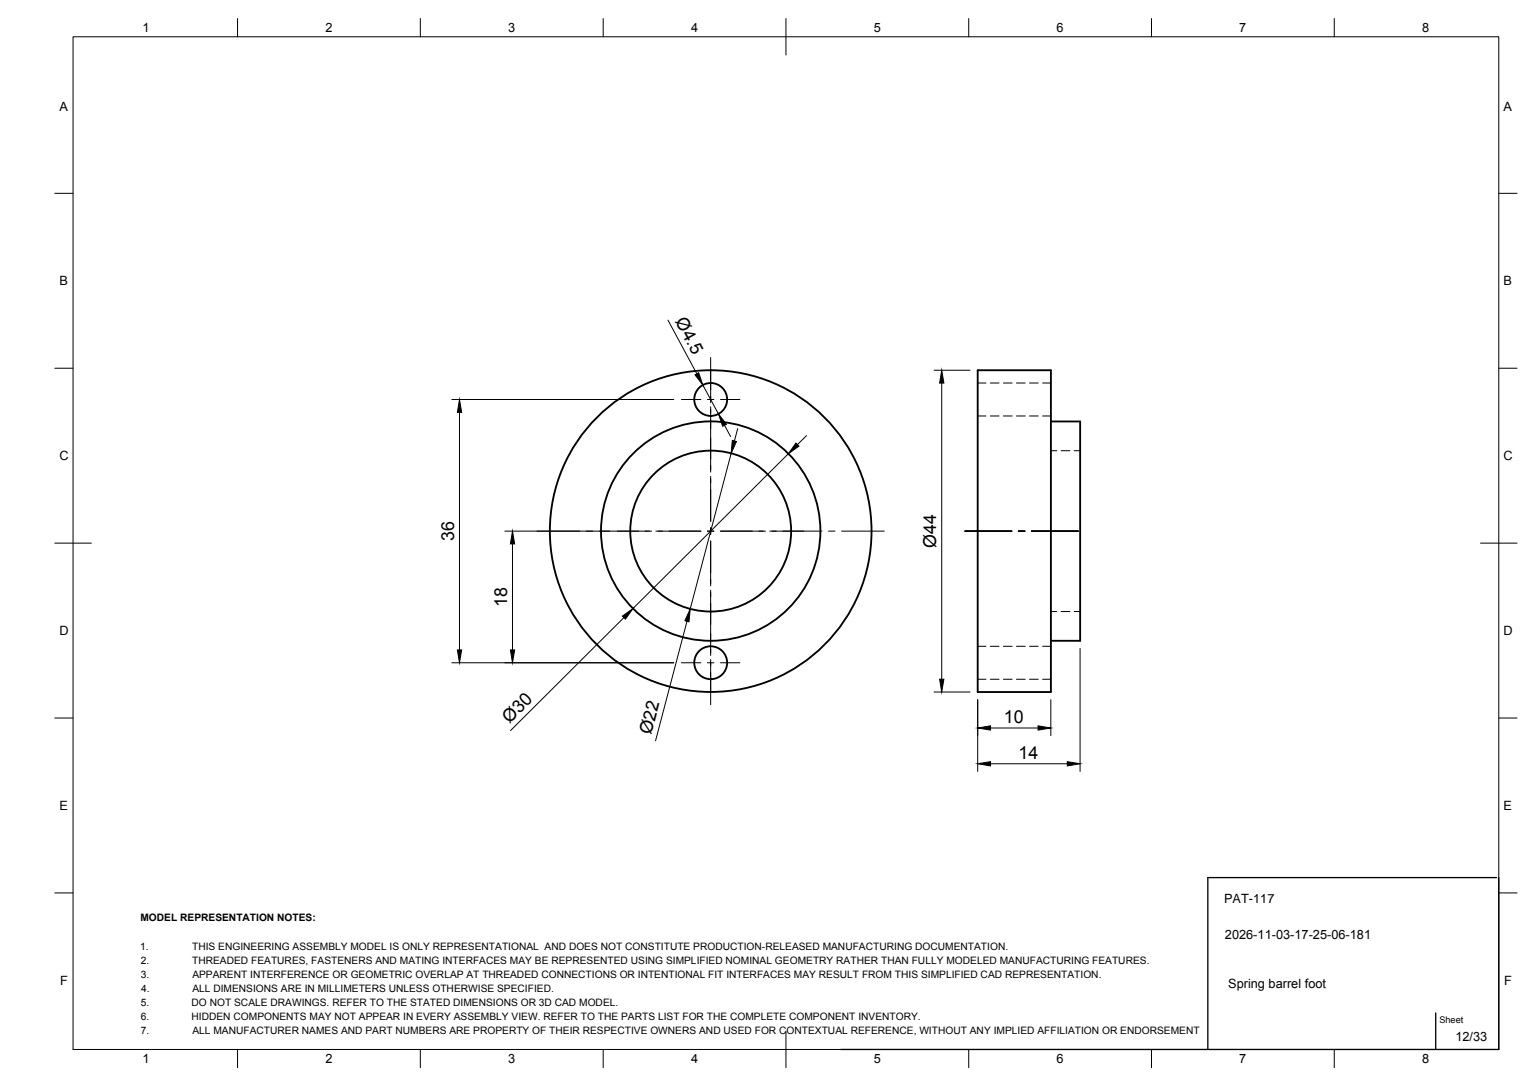
ISO-10303-21;
HEADER;
/* Generated by software containing ST-Developer
 * from STEP Tools, Inc. (www.steptools.com) 
 */

FILE_DESCRIPTION(
/* description */ ('Counterbalanced vertical column'),
/* implementation_level */ '2;1');

FILE_NAME(
/* name */ 'Spring barrel foot.step',
/* time_stamp */ '2026-10-29T16:47:22-07:00',
/* author */ (''),
/* organization */ (''),
/* preprocessor_version */ 'ST-DEVELOPER v20.2',
/* originating_system */ 'Autodesk Translation Framework v15.17.0.0',
/* authorisation */ '');

FILE_SCHEMA (('AUTOMOTIVE_DESIGN { 1 0 10303 214 3 1 1 }'));
ENDSEC;

DATA;
#10=MECHANICAL_DESIGN_GEOMETRIC_PRESENTATION_REPRESENTATION('',(#357),#15040);
#287=SHAPE_REPRESENTATION_RELATIONSHIP('SRR','None',#15191,#322);
#322=ADVANCED_BREP_SHAPE_REPRESENTATION('',(#392),#15010);
#357=STYLED_ITEM('',(#15457),#392);
#392=MANIFOLD_SOLID_BREP('Body1',#7080);
#444=FACE_BOUND('',#1330,.T.);
#445=FACE_BOUND('',#1332,.T.);
#446=FACE_BOUND('',#1333,.T.);
#447=FACE_BOUND('',#1334,.T.);
#448=FACE_BOUND('',#1338,.T.);
#449=FACE_BOUND('',#1339,.T.);
#581=PLANE('',#7618);
#582=PLANE('',#7619);
#583=PLANE('',#7623);
#584=PLANE('',#7624);
#892=FACE_OUTER_BOUND('',#1325,.T.);
#893=FACE_OUTER_BOUND('',#1326,.T.);
#894=FACE_OUTER_BOUND('',#1327,.T.);
#895=FACE_OUTER_BOUND('',#1328,.T.);
#896=FACE_OUTER_BOUND('',#1329,.T.);
#897=FACE_OUTER_BOUND('',#1331,.T.);
#898=FACE_OUTER_BOUND('',#1335,.T.);
#899=FACE_OUTER_BOUND('',#1336,.T.);
#900=FACE_OUTER_BOUND('',#1337,.T.);
#1325=EDGE_LOOP('',(#5076,#5077,#5078,#5079));
#1326=EDGE_LOOP('',(#5080,#5081,#5082,#5083));
#1327=EDGE_LOOP('',(#5084,#5085,#5086,#5087));
#1328=EDGE_LOOP('',(#5088,#5089,#5090,#5091));
#1329=EDGE_LOOP('',(#5092));
#1330=EDGE_LOOP('',(#5093));
#1331=EDGE_LOOP('',(#5094));
#1332=EDGE_LOOP('',(#5095));
#1333=EDGE_LOOP('',(#5096));
#1334=EDGE_LOOP('',(#5097));
#1335=EDGE_LOOP('',(#5098,#5099,#5100,#5101));
#1336=EDGE_LOOP('',(#5102));
#1337=EDGE_LOOP('',(#5103));
#1338=EDGE_LOOP('',(#5104));
#1339=EDGE_LOOP('',(#5105));
#1863=LINE('',#10658,#2534);
#1864=LINE('',#10664,#2535);
#1865=LINE('',#10670,#2536);
#1866=LINE('',#10676,#2537);
#1867=LINE('',#10684,#2538);
#2534=VECTOR('',#8553,0.225);
#2535=VECTOR('',#8560,0.225);
#2536=VECTOR('',#8567,1.1);
#2537=VECTOR('',#8574,1.5);
#2538=VECTOR('',#8585,2.2);
#3125=CIRCLE('',#7607,0.225);
#3126=CIRCLE('',#7608,0.225);
#3127=CIRCLE('',#7610,0.225);
#3128=CIRCLE('',#7611,0.225);
#3129=CIRCLE('',#7613,1.1);
#3130=CIRCLE('',#7614,1.1);
#3131=CIRCLE('',#7616,1.5);
#3132=CIRCLE('',#7617,1.5);
#3133=CIRCLE('',#7620,2.2);
#3134=CIRCLE('',#7622,2.2);
#3402=VERTEX_POINT('',#10655);
#3403=VERTEX_POINT('',#10657);
#3404=VERTEX_POINT('',#10661);
#3405=VERTEX_POINT('',#10663);
#3406=VERTEX_POINT('',#10667);
#3407=VERTEX_POINT('',#10669);
#3408=VERTEX_POINT('',#10673);
#3409=VERTEX_POINT('',#10675);
#3410=VERTEX_POINT('',#10680);
#3411=VERTEX_POINT('',#10683);
#4039=EDGE_CURVE('',#3402,#3402,#3125,.T.);
#4040=EDGE_CURVE('',#3402,#3403,#1863,.T.);
#4041=EDGE_CURVE('',#3403,#3403,#3126,.T.);
#4042=EDGE_CURVE('',#3404,#3404,#3127,.T.);
#4043=EDGE_CURVE('',#3404,#3405,#1864,.T.);
#4044=EDGE_CURVE('',#3405,#3405,#3128,.T.);
#4045=EDGE_CURVE('',#3406,#3406,#3129,.T.);
#4046=EDGE_CURVE('',#3406,#3407,#1865,.T.);
#4047=EDGE_CURVE('',#3407,#3407,#3130,.T.);
#4048=EDGE_CURVE('',#3408,#3408,#3131,.T.);
#4049=EDGE_CURVE('',#3408,#3409,#1866,.T.);
#4050=EDGE_CURVE('',#3409,#3409,#3132,.T.);
#4051=EDGE_CURVE('',#3410,#3410,#3133,.T.);
#4052=EDGE_CURVE('',#3410,#3411,#1867,.T.);
#4053=EDGE_CURVE('',#3411,#3411,#3134,.T.);
#5076=ORIENTED_EDGE('',*,*,#4039,.F.);
#5077=ORIENTED_EDGE('',*,*,#4040,.T.);
#5078=ORIENTED_EDGE('',*,*,#4041,.F.);
#5079=ORIENTED_EDGE('',*,*,#4040,.F.);
#5080=ORIENTED_EDGE('',*,*,#4042,.F.);
#5081=ORIENTED_EDGE('',*,*,#4043,.T.);
#5082=ORIENTED_EDGE('',*,*,#4044,.F.);
#5083=ORIENTED_EDGE('',*,*,#4043,.F.);
#5084=ORIENTED_EDGE('',*,*,#4045,.F.);
#5085=ORIENTED_EDGE('',*,*,#4046,.T.);
#5086=ORIENTED_EDGE('',*,*,#4047,.F.);
#5087=ORIENTED_EDGE('',*,*,#4046,.F.);
#5088=ORIENTED_EDGE('',*,*,#4048,.F.);
#5089=ORIENTED_EDGE('',*,*,#4049,.T.);
#5090=ORIENTED_EDGE('',*,*,#4050,.F.);
#5091=ORIENTED_EDGE('',*,*,#4049,.F.);
#5092=ORIENTED_EDGE('',*,*,#4048,.T.);
#5093=ORIENTED_EDGE('',*,*,#4045,.T.);
#5094=ORIENTED_EDGE('',*,*,#4051,.T.);
#5095=ORIENTED_EDGE('',*,*,#4041,.T.);
#5096=ORIENTED_EDGE('',*,*,#4044,.T.);
#5097=ORIENTED_EDGE('',*,*,#4050,.T.);
#5098=ORIENTED_EDGE('',*,*,#4051,.F.);
#5099=ORIENTED_EDGE('',*,*,#4052,.T.);
#5100=ORIENTED_EDGE('',*,*,#4053,.T.);
#5101=ORIENTED_EDGE('',*,*,#4052,.F.);
#5102=ORIENTED_EDGE('',*,*,#4047,.T.);
#5103=ORIENTED_EDGE('',*,*,#4053,.F.);
#5104=ORIENTED_EDGE('',*,*,#4039,.T.);
#5105=ORIENTED_EDGE('',*,*,#4042,.T.);
#6590=CYLINDRICAL_SURFACE('',#7606,0.225);
#6591=CYLINDRICAL_SURFACE('',#7609,0.225);
#6592=CYLINDRICAL_SURFACE('',#7612,1.1);
#6593=CYLINDRICAL_SURFACE('',#7615,1.5);
#6594=CYLINDRICAL_SURFACE('',#7621,2.2);
#6734=ADVANCED_FACE('',(#892),#6590,.F.);
#6735=ADVANCED_FACE('',(#893),#6591,.F.);
#6736=ADVANCED_FACE('',(#894),#6592,.F.);
#6737=ADVANCED_FACE('',(#895),#6593,.T.);
#6738=ADVANCED_FACE('',(#896,#444),#581,.T.);
#6739=ADVANCED_FACE('',(#897,#445,#446,#447),#582,.T.);
#6740=ADVANCED_FACE('',(#898),#6594,.T.);
#6741=ADVANCED_FACE('',(#899),#583,.T.);
#6742=ADVANCED_FACE('',(#900,#448,#449),#584,.F.);
#7080=CLOSED_SHELL('',(#6734,#6735,#6736,#6737,#6738,#6739,#6740,#6741,
#6742));
#7605=AXIS2_PLACEMENT_3D('',#10653,#8547,#8548);
#7606=AXIS2_PLACEMENT_3D('',#10654,#8549,#8550);
#7607=AXIS2_PLACEMENT_3D('',#10656,#8551,#8552);
#7608=AXIS2_PLACEMENT_3D('',#10659,#8554,#8555);
#7609=AXIS2_PLACEMENT_3D('',#10660,#8556,#8557);
#7610=AXIS2_PLACEMENT_3D('',#10662,#8558,#8559);
#7611=AXIS2_PLACEMENT_3D('',#10665,#8561,#8562);
#7612=AXIS2_PLACEMENT_3D('',#10666,#8563,#8564);
#7613=AXIS2_PLACEMENT_3D('',#10668,#8565,#8566);
#7614=AXIS2_PLACEMENT_3D('',#10671,#8568,#8569);
#7615=AXIS2_PLACEMENT_3D('',#10672,#8570,#8571);
#7616=AXIS2_PLACEMENT_3D('',#10674,#8572,#8573);
#7617=AXIS2_PLACEMENT_3D('',#10677,#8575,#8576);
#7618=AXIS2_PLACEMENT_3D('',#10678,#8577,#8578);
#7619=AXIS2_PLACEMENT_3D('',#10679,#8579,#8580);
#7620=AXIS2_PLACEMENT_3D('',#10681,#8581,#8582);
#7621=AXIS2_PLACEMENT_3D('',#10682,#8583,#8584);
#7622=AXIS2_PLACEMENT_3D('',#10685,#8586,#8587);
#7623=AXIS2_PLACEMENT_3D('',#10686,#8588,#8589);
#7624=AXIS2_PLACEMENT_3D('',#10687,#8590,#8591);
#8547=DIRECTION('axis',(0.,0.,1.));
#8548=DIRECTION('refdir',(1.,0.,0.));
#8549=DIRECTION('center_axis',(0.,0.,1.));
#8550=DIRECTION('ref_axis',(1.,0.,0.));
#8551=DIRECTION('center_axis',(0.,0.,1.));
#8552=DIRECTION('ref_axis',(1.,0.,0.));
#8553=DIRECTION('',(0.,0.,1.));
#8554=DIRECTION('center_axis',(0.,0.,-1.));
#8555=DIRECTION('ref_axis',(1.,0.,0.));
#8556=DIRECTION('center_axis',(0.,0.,1.));
#8557=DIRECTION('ref_axis',(1.,0.,0.));
#8558=DIRECTION('center_axis',(0.,0.,1.));
#8559=DIRECTION('ref_axis',(1.,0.,0.));
#8560=DIRECTION('',(0.,0.,1.));
#8561=DIRECTION('center_axis',(0.,0.,-1.));
#8562=DIRECTION('ref_axis',(1.,0.,0.));
#8563=DIRECTION('center_axis',(0.,0.,1.));
#8564=DIRECTION('ref_axis',(1.,0.,0.));
#8565=DIRECTION('center_axis',(0.,0.,-1.));
#8566=DIRECTION('ref_axis',(1.,0.,0.));
#8567=DIRECTION('',(0.,0.,-1.));
#8568=DIRECTION('center_axis',(0.,0.,1.));
#8569=DIRECTION('ref_axis',(1.,0.,0.));
#8570=DIRECTION('center_axis',(0.,0.,1.));
#8571=DIRECTION('ref_axis',(1.,0.,0.));
#8572=DIRECTION('center_axis',(0.,0.,1.));
#8573=DIRECTION('ref_axis',(1.,0.,0.));
#8574=DIRECTION('',(0.,0.,-1.));
#8575=DIRECTION('center_axis',(0.,0.,-1.));
#8576=DIRECTION('ref_axis',(1.,0.,0.));
#8577=DIRECTION('center_axis',(0.,0.,1.));
#8578=DIRECTION('ref_axis',(1.,0.,0.));
#8579=DIRECTION('center_axis',(0.,0.,1.));
#8580=DIRECTION('ref_axis',(1.,0.,0.));
#8581=DIRECTION('center_axis',(0.,0.,1.));
#8582=DIRECTION('ref_axis',(1.,0.,0.));
#8583=DIRECTION('center_axis',(0.,0.,1.));
#8584=DIRECTION('ref_axis',(1.,0.,0.));
#8585=DIRECTION('',(0.,0.,-1.));
#8586=DIRECTION('center_axis',(0.,0.,1.));
#8587=DIRECTION('ref_axis',(1.,0.,0.));
#8588=DIRECTION('center_axis',(0.,0.,1.));
#8589=DIRECTION('ref_axis',(1.,0.,0.));
#8590=DIRECTION('center_axis',(0.,0.,1.));
#8591=DIRECTION('ref_axis',(1.,0.,0.));
#10653=CARTESIAN_POINT('',(0.,0.,0.));
#10654=CARTESIAN_POINT('Origin',(-5.2,0.,-0.1));
#10655=CARTESIAN_POINT('',(-5.425,-2.75545529808154E-17,0.));
#10656=CARTESIAN_POINT('Origin',(-5.2,0.,0.));
#10657=CARTESIAN_POINT('',(-5.425,2.75545529808154E-17,1.));
#10658=CARTESIAN_POINT('',(-5.425,-2.75545529808154E-17,-0.1));
#10659=CARTESIAN_POINT('Origin',(-5.2,0.,1.));
#10660=CARTESIAN_POINT('Origin',(-8.8,0.,-0.1));
#10661=CARTESIAN_POINT('',(-9.025,-2.75545529808154E-17,0.));
#10662=CARTESIAN_POINT('Origin',(-8.8,0.,0.));
#10663=CARTESIAN_POINT('',(-9.025,2.75545529808154E-17,1.));
#10664=CARTESIAN_POINT('',(-9.025,-2.75545529808154E-17,-0.1));
#10665=CARTESIAN_POINT('Origin',(-8.8,0.,1.));
#10666=CARTESIAN_POINT('Origin',(-7.,0.,1.));
#10667=CARTESIAN_POINT('',(-8.1,-1.34711147906209E-16,1.4));
#10668=CARTESIAN_POINT('Origin',(-7.,0.,1.4));
#10669=CARTESIAN_POINT('',(-8.1,-1.34711147906209E-16,1.));
#10670=CARTESIAN_POINT('',(-8.1,-1.34711147906209E-16,1.));
#10671=CARTESIAN_POINT('Origin',(-7.,0.,1.));
#10672=CARTESIAN_POINT('Origin',(-7.,0.,1.));
#10673=CARTESIAN_POINT('',(-8.5,-1.83697019872103E-16,1.4));
#10674=CARTESIAN_POINT('Origin',(-7.,0.,1.4));
#10675=CARTESIAN_POINT('',(-8.5,-1.83697019872103E-16,1.));
#10676=CARTESIAN_POINT('',(-8.5,-1.83697019872103E-16,1.));
#10677=CARTESIAN_POINT('Origin',(-7.,0.,1.));
#10678=CARTESIAN_POINT('Origin',(-7.,0.,1.4));
#10679=CARTESIAN_POINT('Origin',(-7.,0.,1.));
#10680=CARTESIAN_POINT('',(-9.2,-2.69422295812418E-16,1.));
#10681=CARTESIAN_POINT('Origin',(-7.,0.,1.));
#10682=CARTESIAN_POINT('Origin',(-7.,0.,0.));
#10683=CARTESIAN_POINT('',(-9.2,-2.69422295812418E-16,0.));
#10684=CARTESIAN_POINT('',(-9.2,-2.69422295812418E-16,0.));
#10685=CARTESIAN_POINT('Origin',(-7.,0.,0.));
#10686=CARTESIAN_POINT('Origin',(-7.,0.,1.));
#10687=CARTESIAN_POINT('Origin',(-7.,0.,0.));
#14970=UNCERTAINTY_MEASURE_WITH_UNIT(LENGTH_MEASURE(0.001),#15041,
'DISTANCE_ACCURACY_VALUE',
'Maximum model space distance between geometric entities at asserted c
onnectivities');
#15000=UNCERTAINTY_MEASURE_WITH_UNIT(LENGTH_MEASURE(0.001),#15041,
'DISTANCE_ACCURACY_VALUE',
'Maximum model space distance between geometric entities at asserted c
onnectivities');
#15010=(
GEOMETRIC_REPRESENTATION_CONTEXT(3)
GLOBAL_UNCERTAINTY_ASSIGNED_CONTEXT((#14970))
GLOBAL_UNIT_ASSIGNED_CONTEXT((#15041,#15043,#15044))
REPRESENTATION_CONTEXT('','3D')
);
#15040=(
GEOMETRIC_REPRESENTATION_CONTEXT(3)
GLOBAL_UNCERTAINTY_ASSIGNED_CONTEXT((#15000))
GLOBAL_UNIT_ASSIGNED_CONTEXT((#15041,#15043,#15044))
REPRESENTATION_CONTEXT('','3D')
);
#15041=(
LENGTH_UNIT()
NAMED_UNIT(*)
SI_UNIT(.CENTI.,.METRE.)
);
#15043=(
NAMED_UNIT(*)
PLANE_ANGLE_UNIT()
SI_UNIT($,.RADIAN.)
);
#15044=(
NAMED_UNIT(*)
SI_UNIT($,.STERADIAN.)
SOLID_ANGLE_UNIT()
);
#15054=SHAPE_DEFINITION_REPRESENTATION(#15093,#15191);
#15093=PRODUCT_DEFINITION_SHAPE('',$,#15231);
#15191=SHAPE_REPRESENTATION('',(#7605),#15010);
#15221=PRODUCT_DEFINITION_CONTEXT('part definition',#15340,'design');
#15231=PRODUCT_DEFINITION('Spring barrel foot','Spring barrel foot',#15270,
#15221);
#15270=PRODUCT_DEFINITION_FORMATION('',$,#15351);
#15340=APPLICATION_CONTEXT(
'Core Data for Automotive Mechanical Design Process');
#15341=PRODUCT_CONTEXT('part definition',#15340,'mechanical');
#15351=PRODUCT('Spring barrel foot','Spring barrel foot',
'Spring barrel foot',(#15341));
#15451=COLOUR_RGB('Grey',0.48,0.52,0.57);
#15452=FILL_AREA_STYLE_COLOUR('',#15451);
#15453=FILL_AREA_STYLE('',(#15452));
#15454=SURFACE_STYLE_FILL_AREA(#15453);
#15455=SURFACE_SIDE_STYLE('',(#15454));
#15456=SURFACE_STYLE_USAGE(.BOTH.,#15455);
#15457=PRESENTATION_STYLE_ASSIGNMENT((#15456));
ENDSEC;
END-ISO-10303-21;
